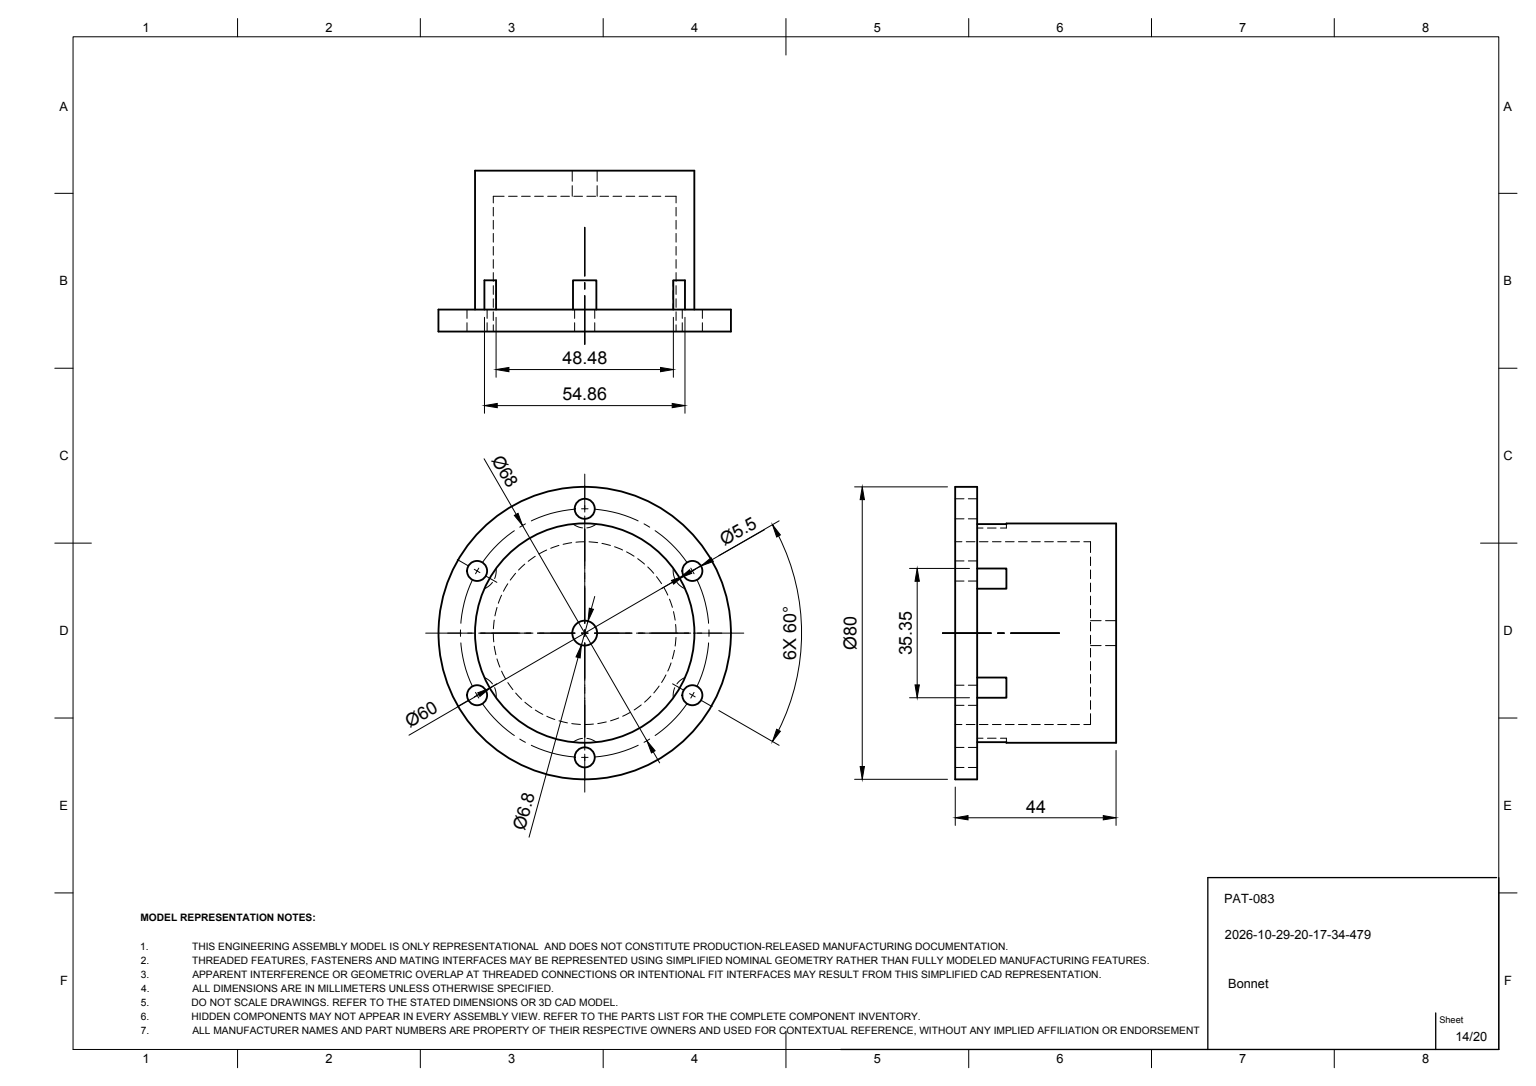
ISO-10303-21;
HEADER;
/* Generated by software containing ST-Developer
 * from STEP Tools, Inc. (www.steptools.com) 
 */

FILE_DESCRIPTION(
/* description */ ('PAT-083'),
/* implementation_level */ '2;1');

FILE_NAME(
/* name */ 'Bonnet.step',
/* time_stamp */ '2026-10-29T20:18:00-07:00',
/* author */ (''),
/* organization */ (''),
/* preprocessor_version */ 'ST-DEVELOPER v20.2',
/* originating_system */ 'Autodesk Translation Framework v15.17.0.0',
/* authorisation */ '');

FILE_SCHEMA (('AUTOMOTIVE_DESIGN { 1 0 10303 214 3 1 1 }'));
ENDSEC;

DATA;
#10=MECHANICAL_DESIGN_GEOMETRIC_PRESENTATION_REPRESENTATION('',(#240),#8428);
#192=SHAPE_REPRESENTATION_RELATIONSHIP('SRR','None',#8526,#216);
#216=ADVANCED_BREP_SHAPE_REPRESENTATION('',(#264),#8415);
#240=STYLED_ITEM('',(#8698),#264);
#264=MANIFOLD_SOLID_BREP('Body1',#3686);
#324=FACE_BOUND('',#900,.T.);
#325=FACE_BOUND('',#902,.T.);
#326=FACE_BOUND('',#905,.T.);
#327=FACE_BOUND('',#906,.T.);
#328=FACE_BOUND('',#907,.T.);
#329=FACE_BOUND('',#908,.T.);
#330=FACE_BOUND('',#909,.T.);
#331=FACE_BOUND('',#910,.T.);
#332=FACE_BOUND('',#911,.T.);
#333=FACE_BOUND('',#913,.T.);
#334=FACE_BOUND('',#914,.T.);
#335=FACE_BOUND('',#915,.T.);
#336=FACE_BOUND('',#916,.T.);
#337=FACE_BOUND('',#917,.T.);
#338=FACE_BOUND('',#918,.T.);
#339=FACE_BOUND('',#919,.T.);
#411=PLANE('',#4167);
#412=PLANE('',#4175);
#413=PLANE('',#4177);
#414=PLANE('',#4182);
#415=PLANE('',#4187);
#416=PLANE('',#4195);
#417=PLANE('',#4230);
#418=PLANE('',#4231);
#419=PLANE('',#4235);
#420=PLANE('',#4236);
#596=FACE_OUTER_BOUND('',#878,.T.);
#597=FACE_OUTER_BOUND('',#879,.T.);
#598=FACE_OUTER_BOUND('',#880,.T.);
#599=FACE_OUTER_BOUND('',#881,.T.);
#600=FACE_OUTER_BOUND('',#882,.T.);
#601=FACE_OUTER_BOUND('',#883,.T.);
#602=FACE_OUTER_BOUND('',#884,.T.);
#603=FACE_OUTER_BOUND('',#885,.T.);
#604=FACE_OUTER_BOUND('',#886,.T.);
#605=FACE_OUTER_BOUND('',#887,.T.);
#606=FACE_OUTER_BOUND('',#888,.T.);
#607=FACE_OUTER_BOUND('',#889,.T.);
#608=FACE_OUTER_BOUND('',#890,.T.);
#609=FACE_OUTER_BOUND('',#891,.T.);
#610=FACE_OUTER_BOUND('',#892,.T.);
#611=FACE_OUTER_BOUND('',#893,.T.);
#612=FACE_OUTER_BOUND('',#894,.T.);
#613=FACE_OUTER_BOUND('',#895,.T.);
#614=FACE_OUTER_BOUND('',#896,.T.);
#615=FACE_OUTER_BOUND('',#897,.T.);
#616=FACE_OUTER_BOUND('',#898,.T.);
#617=FACE_OUTER_BOUND('',#899,.T.);
#618=FACE_OUTER_BOUND('',#901,.T.);
#619=FACE_OUTER_BOUND('',#903,.T.);
#620=FACE_OUTER_BOUND('',#904,.T.);
#621=FACE_OUTER_BOUND('',#912,.T.);
#878=EDGE_LOOP('',(#2828,#2829));
#879=EDGE_LOOP('',(#2830,#2831,#2832,#2833));
#880=EDGE_LOOP('',(#2834,#2835,#2836,#2837));
#881=EDGE_LOOP('',(#2838,#2839));
#882=EDGE_LOOP('',(#2840,#2841));
#883=EDGE_LOOP('',(#2842,#2843,#2844,#2845));
#884=EDGE_LOOP('',(#2846,#2847));
#885=EDGE_LOOP('',(#2848,#2849,#2850,#2851));
#886=EDGE_LOOP('',(#2852,#2853));
#887=EDGE_LOOP('',(#2854,#2855,#2856,#2857));
#888=EDGE_LOOP('',(#2858,#2859,#2860,#2861));
#889=EDGE_LOOP('',(#2862,#2863));
#890=EDGE_LOOP('',(#2864,#2865,#2866,#2867,#2868,#2869,#2870,#2871,#2872,
#2873,#2874,#2875,#2876,#2877,#2878,#2879,#2880,#2881,#2882,#2883,#2884,
#2885,#2886,#2887,#2888,#2889,#2890,#2891));
#891=EDGE_LOOP('',(#2892,#2893,#2894,#2895));
#892=EDGE_LOOP('',(#2896,#2897,#2898,#2899));
#893=EDGE_LOOP('',(#2900,#2901,#2902,#2903));
#894=EDGE_LOOP('',(#2904,#2905,#2906,#2907));
#895=EDGE_LOOP('',(#2908,#2909,#2910,#2911));
#896=EDGE_LOOP('',(#2912,#2913,#2914,#2915));
#897=EDGE_LOOP('',(#2916,#2917,#2918,#2919));
#898=EDGE_LOOP('',(#2920,#2921,#2922,#2923));
#899=EDGE_LOOP('',(#2924));
#900=EDGE_LOOP('',(#2925));
#901=EDGE_LOOP('',(#2926));
#902=EDGE_LOOP('',(#2927));
#903=EDGE_LOOP('',(#2928,#2929,#2930,#2931));
#904=EDGE_LOOP('',(#2932));
#905=EDGE_LOOP('',(#2933));
#906=EDGE_LOOP('',(#2934));
#907=EDGE_LOOP('',(#2935));
#908=EDGE_LOOP('',(#2936));
#909=EDGE_LOOP('',(#2937));
#910=EDGE_LOOP('',(#2938));
#911=EDGE_LOOP('',(#2939,#2940,#2941,#2942,#2943,#2944,#2945,#2946,#2947,
#2948,#2949,#2950,#2951));
#912=EDGE_LOOP('',(#2952));
#913=EDGE_LOOP('',(#2953));
#914=EDGE_LOOP('',(#2954));
#915=EDGE_LOOP('',(#2955));
#916=EDGE_LOOP('',(#2956));
#917=EDGE_LOOP('',(#2957));
#918=EDGE_LOOP('',(#2958));
#919=EDGE_LOOP('',(#2959));
#1129=LINE('',#6913,#1373);
#1130=LINE('',#6916,#1374);
#1131=LINE('',#6920,#1375);
#1132=LINE('',#6924,#1376);
#1133=LINE('',#6935,#1377);
#1134=LINE('',#6938,#1378);
#1135=LINE('',#6946,#1379);
#1136=LINE('',#6949,#1380);
#1137=LINE('',#6957,#1381);
#1138=LINE('',#6960,#1382);
#1139=LINE('',#6964,#1383);
#1140=LINE('',#6968,#1384);
#1141=LINE('',#6976,#1385);
#1142=LINE('',#6988,#1386);
#1143=LINE('',#6994,#1387);
#1144=LINE('',#7000,#1388);
#1145=LINE('',#7006,#1389);
#1146=LINE('',#7012,#1390);
#1147=LINE('',#7018,#1391);
#1148=LINE('',#7024,#1392);
#1149=LINE('',#7030,#1393);
#1150=LINE('',#7038,#1394);
#1373=VECTOR('',#4933,1.);
#1374=VECTOR('',#4936,1.);
#1375=VECTOR('',#4939,1.);
#1376=VECTOR('',#4942,1.);
#1377=VECTOR('',#4957,1.);
#1378=VECTOR('',#4960,1.);
#1379=VECTOR('',#4969,1.);
#1380=VECTOR('',#4972,1.);
#1381=VECTOR('',#4981,1.);
#1382=VECTOR('',#4984,1.);
#1383=VECTOR('',#4987,1.);
#1384=VECTOR('',#4990,1.);
#1385=VECTOR('',#5001,3.);
#1386=VECTOR('',#5020,0.275);
#1387=VECTOR('',#5027,0.275);
#1388=VECTOR('',#5034,0.275);
#1389=VECTOR('',#5041,0.275);
#1390=VECTOR('',#5048,0.275);
#1391=VECTOR('',#5055,0.275);
#1392=VECTOR('',#5062,0.34);
#1393=VECTOR('',#5069,2.5);
#1394=VECTOR('',#5080,4.);
#1618=CIRCLE('',#4168,3.);
#1619=CIRCLE('',#4169,0.525);
#1620=CIRCLE('',#4171,0.525);
#1621=CIRCLE('',#4173,0.525);
#1622=CIRCLE('',#4174,0.525);
#1623=CIRCLE('',#4176,3.);
#1624=CIRCLE('',#4178,3.);
#1625=CIRCLE('',#4179,0.525);
#1626=CIRCLE('',#4181,0.525);
#1627=CIRCLE('',#4183,3.);
#1628=CIRCLE('',#4184,0.525);
#1629=CIRCLE('',#4186,0.525);
#1630=CIRCLE('',#4188,3.);
#1631=CIRCLE('',#4189,0.525);
#1632=CIRCLE('',#4191,0.525);
#1633=CIRCLE('',#4193,0.525);
#1634=CIRCLE('',#4194,0.525);
#1635=CIRCLE('',#4196,3.);
#1636=CIRCLE('',#4198,3.);
#1637=CIRCLE('',#4199,3.);
#1638=CIRCLE('',#4200,3.);
#1639=CIRCLE('',#4201,3.);
#1640=CIRCLE('',#4202,3.);
#1641=CIRCLE('',#4203,3.);
#1642=CIRCLE('',#4204,3.);
#1643=CIRCLE('',#4205,3.);
#1644=CIRCLE('',#4207,0.275);
#1645=CIRCLE('',#4208,0.275);
#1646=CIRCLE('',#4210,0.275);
#1647=CIRCLE('',#4211,0.275);
#1648=CIRCLE('',#4213,0.275);
#1649=CIRCLE('',#4214,0.275);
#1650=CIRCLE('',#4216,0.275);
#1651=CIRCLE('',#4217,0.275);
#1652=CIRCLE('',#4219,0.275);
#1653=CIRCLE('',#4220,0.275);
#1654=CIRCLE('',#4222,0.275);
#1655=CIRCLE('',#4223,0.275);
#1656=CIRCLE('',#4225,0.34);
#1657=CIRCLE('',#4226,0.34);
#1658=CIRCLE('',#4228,2.5);
#1659=CIRCLE('',#4229,2.5);
#1660=CIRCLE('',#4233,4.);
#1661=CIRCLE('',#4234,4.);
#1831=VERTEX_POINT('',#6907);
#1832=VERTEX_POINT('',#6908);
#1833=VERTEX_POINT('',#6912);
#1834=VERTEX_POINT('',#6914);
#1835=VERTEX_POINT('',#6918);
#1836=VERTEX_POINT('',#6919);
#1837=VERTEX_POINT('',#6921);
#1838=VERTEX_POINT('',#6923);
#1839=VERTEX_POINT('',#6929);
#1840=VERTEX_POINT('',#6930);
#1841=VERTEX_POINT('',#6934);
#1842=VERTEX_POINT('',#6936);
#1843=VERTEX_POINT('',#6940);
#1844=VERTEX_POINT('',#6941);
#1845=VERTEX_POINT('',#6945);
#1846=VERTEX_POINT('',#6947);
#1847=VERTEX_POINT('',#6951);
#1848=VERTEX_POINT('',#6952);
#1849=VERTEX_POINT('',#6956);
#1850=VERTEX_POINT('',#6958);
#1851=VERTEX_POINT('',#6962);
#1852=VERTEX_POINT('',#6963);
#1853=VERTEX_POINT('',#6965);
#1854=VERTEX_POINT('',#6967);
#1855=VERTEX_POINT('',#6973);
#1856=VERTEX_POINT('',#6975);
#1857=VERTEX_POINT('',#6985);
#1858=VERTEX_POINT('',#6987);
#1859=VERTEX_POINT('',#6991);
#1860=VERTEX_POINT('',#6993);
#1861=VERTEX_POINT('',#6997);
#1862=VERTEX_POINT('',#6999);
#1863=VERTEX_POINT('',#7003);
#1864=VERTEX_POINT('',#7005);
#1865=VERTEX_POINT('',#7009);
#1866=VERTEX_POINT('',#7011);
#1867=VERTEX_POINT('',#7015);
#1868=VERTEX_POINT('',#7017);
#1869=VERTEX_POINT('',#7021);
#1870=VERTEX_POINT('',#7023);
#1871=VERTEX_POINT('',#7027);
#1872=VERTEX_POINT('',#7029);
#1873=VERTEX_POINT('',#7035);
#1874=VERTEX_POINT('',#7037);
#2190=EDGE_CURVE('',#1831,#1832,#1618,.T.);
#2191=EDGE_CURVE('',#1832,#1831,#1619,.T.);
#2192=EDGE_CURVE('',#1833,#1831,#1129,.T.);
#2193=EDGE_CURVE('',#1834,#1833,#1620,.T.);
#2194=EDGE_CURVE('',#1832,#1834,#1130,.T.);
#2195=EDGE_CURVE('',#1835,#1836,#1131,.T.);
#2196=EDGE_CURVE('',#1835,#1837,#1621,.T.);
#2197=EDGE_CURVE('',#1838,#1837,#1132,.T.);
#2198=EDGE_CURVE('',#1836,#1838,#1622,.T.);
#2199=EDGE_CURVE('',#1837,#1835,#1623,.T.);
#2200=EDGE_CURVE('',#1839,#1840,#1624,.T.);
#2201=EDGE_CURVE('',#1840,#1839,#1625,.T.);
#2202=EDGE_CURVE('',#1841,#1839,#1133,.T.);
#2203=EDGE_CURVE('',#1842,#1841,#1626,.T.);
#2204=EDGE_CURVE('',#1840,#1842,#1134,.T.);
#2205=EDGE_CURVE('',#1843,#1844,#1627,.T.);
#2206=EDGE_CURVE('',#1844,#1843,#1628,.T.);
#2207=EDGE_CURVE('',#1845,#1843,#1135,.T.);
#2208=EDGE_CURVE('',#1846,#1845,#1629,.T.);
#2209=EDGE_CURVE('',#1844,#1846,#1136,.T.);
#2210=EDGE_CURVE('',#1847,#1848,#1630,.T.);
#2211=EDGE_CURVE('',#1848,#1847,#1631,.T.);
#2212=EDGE_CURVE('',#1849,#1847,#1137,.T.);
#2213=EDGE_CURVE('',#1850,#1849,#1632,.T.);
#2214=EDGE_CURVE('',#1848,#1850,#1138,.T.);
#2215=EDGE_CURVE('',#1851,#1852,#1139,.T.);
#2216=EDGE_CURVE('',#1851,#1853,#1633,.T.);
#2217=EDGE_CURVE('',#1854,#1853,#1140,.T.);
#2218=EDGE_CURVE('',#1852,#1854,#1634,.T.);
#2219=EDGE_CURVE('',#1853,#1851,#1635,.T.);
#2220=EDGE_CURVE('',#1855,#1855,#1636,.T.);
#2221=EDGE_CURVE('',#1855,#1856,#1141,.T.);
#2222=EDGE_CURVE('',#1849,#1856,#1637,.T.);
#2223=EDGE_CURVE('',#1833,#1850,#1638,.T.);
#2224=EDGE_CURVE('',#1854,#1834,#1639,.T.);
#2225=EDGE_CURVE('',#1838,#1852,#1640,.T.);
#2226=EDGE_CURVE('',#1841,#1836,#1641,.T.);
#2227=EDGE_CURVE('',#1845,#1842,#1642,.T.);
#2228=EDGE_CURVE('',#1856,#1846,#1643,.T.);
#2229=EDGE_CURVE('',#1857,#1857,#1644,.T.);
#2230=EDGE_CURVE('',#1857,#1858,#1142,.T.);
#2231=EDGE_CURVE('',#1858,#1858,#1645,.T.);
#2232=EDGE_CURVE('',#1859,#1859,#1646,.T.);
#2233=EDGE_CURVE('',#1859,#1860,#1143,.T.);
#2234=EDGE_CURVE('',#1860,#1860,#1647,.T.);
#2235=EDGE_CURVE('',#1861,#1861,#1648,.T.);
#2236=EDGE_CURVE('',#1861,#1862,#1144,.T.);
#2237=EDGE_CURVE('',#1862,#1862,#1649,.T.);
#2238=EDGE_CURVE('',#1863,#1863,#1650,.T.);
#2239=EDGE_CURVE('',#1863,#1864,#1145,.T.);
#2240=EDGE_CURVE('',#1864,#1864,#1651,.T.);
#2241=EDGE_CURVE('',#1865,#1865,#1652,.T.);
#2242=EDGE_CURVE('',#1865,#1866,#1146,.T.);
#2243=EDGE_CURVE('',#1866,#1866,#1653,.T.);
#2244=EDGE_CURVE('',#1867,#1867,#1654,.T.);
#2245=EDGE_CURVE('',#1867,#1868,#1147,.T.);
#2246=EDGE_CURVE('',#1868,#1868,#1655,.T.);
#2247=EDGE_CURVE('',#1869,#1869,#1656,.T.);
#2248=EDGE_CURVE('',#1869,#1870,#1148,.T.);
#2249=EDGE_CURVE('',#1870,#1870,#1657,.T.);
#2250=EDGE_CURVE('',#1871,#1871,#1658,.T.);
#2251=EDGE_CURVE('',#1871,#1872,#1149,.T.);
#2252=EDGE_CURVE('',#1872,#1872,#1659,.T.);
#2253=EDGE_CURVE('',#1873,#1873,#1660,.T.);
#2254=EDGE_CURVE('',#1873,#1874,#1150,.T.);
#2255=EDGE_CURVE('',#1874,#1874,#1661,.T.);
#2828=ORIENTED_EDGE('',*,*,#2190,.F.);
#2829=ORIENTED_EDGE('',*,*,#2191,.F.);
#2830=ORIENTED_EDGE('',*,*,#2192,.F.);
#2831=ORIENTED_EDGE('',*,*,#2193,.F.);
#2832=ORIENTED_EDGE('',*,*,#2194,.F.);
#2833=ORIENTED_EDGE('',*,*,#2191,.T.);
#2834=ORIENTED_EDGE('',*,*,#2195,.F.);
#2835=ORIENTED_EDGE('',*,*,#2196,.T.);
#2836=ORIENTED_EDGE('',*,*,#2197,.F.);
#2837=ORIENTED_EDGE('',*,*,#2198,.F.);
#2838=ORIENTED_EDGE('',*,*,#2199,.F.);
#2839=ORIENTED_EDGE('',*,*,#2196,.F.);
#2840=ORIENTED_EDGE('',*,*,#2200,.F.);
#2841=ORIENTED_EDGE('',*,*,#2201,.F.);
#2842=ORIENTED_EDGE('',*,*,#2202,.F.);
#2843=ORIENTED_EDGE('',*,*,#2203,.F.);
#2844=ORIENTED_EDGE('',*,*,#2204,.F.);
#2845=ORIENTED_EDGE('',*,*,#2201,.T.);
#2846=ORIENTED_EDGE('',*,*,#2205,.F.);
#2847=ORIENTED_EDGE('',*,*,#2206,.F.);
#2848=ORIENTED_EDGE('',*,*,#2207,.F.);
#2849=ORIENTED_EDGE('',*,*,#2208,.F.);
#2850=ORIENTED_EDGE('',*,*,#2209,.F.);
#2851=ORIENTED_EDGE('',*,*,#2206,.T.);
#2852=ORIENTED_EDGE('',*,*,#2210,.F.);
#2853=ORIENTED_EDGE('',*,*,#2211,.F.);
#2854=ORIENTED_EDGE('',*,*,#2212,.F.);
#2855=ORIENTED_EDGE('',*,*,#2213,.F.);
#2856=ORIENTED_EDGE('',*,*,#2214,.F.);
#2857=ORIENTED_EDGE('',*,*,#2211,.T.);
#2858=ORIENTED_EDGE('',*,*,#2215,.F.);
#2859=ORIENTED_EDGE('',*,*,#2216,.T.);
#2860=ORIENTED_EDGE('',*,*,#2217,.F.);
#2861=ORIENTED_EDGE('',*,*,#2218,.F.);
#2862=ORIENTED_EDGE('',*,*,#2219,.F.);
#2863=ORIENTED_EDGE('',*,*,#2216,.F.);
#2864=ORIENTED_EDGE('',*,*,#2220,.F.);
#2865=ORIENTED_EDGE('',*,*,#2221,.T.);
#2866=ORIENTED_EDGE('',*,*,#2222,.F.);
#2867=ORIENTED_EDGE('',*,*,#2212,.T.);
#2868=ORIENTED_EDGE('',*,*,#2210,.T.);
#2869=ORIENTED_EDGE('',*,*,#2214,.T.);
#2870=ORIENTED_EDGE('',*,*,#2223,.F.);
#2871=ORIENTED_EDGE('',*,*,#2192,.T.);
#2872=ORIENTED_EDGE('',*,*,#2190,.T.);
#2873=ORIENTED_EDGE('',*,*,#2194,.T.);
#2874=ORIENTED_EDGE('',*,*,#2224,.F.);
#2875=ORIENTED_EDGE('',*,*,#2217,.T.);
#2876=ORIENTED_EDGE('',*,*,#2219,.T.);
#2877=ORIENTED_EDGE('',*,*,#2215,.T.);
#2878=ORIENTED_EDGE('',*,*,#2225,.F.);
#2879=ORIENTED_EDGE('',*,*,#2197,.T.);
#2880=ORIENTED_EDGE('',*,*,#2199,.T.);
#2881=ORIENTED_EDGE('',*,*,#2195,.T.);
#2882=ORIENTED_EDGE('',*,*,#2226,.F.);
#2883=ORIENTED_EDGE('',*,*,#2202,.T.);
#2884=ORIENTED_EDGE('',*,*,#2200,.T.);
#2885=ORIENTED_EDGE('',*,*,#2204,.T.);
#2886=ORIENTED_EDGE('',*,*,#2227,.F.);
#2887=ORIENTED_EDGE('',*,*,#2207,.T.);
#2888=ORIENTED_EDGE('',*,*,#2205,.T.);
#2889=ORIENTED_EDGE('',*,*,#2209,.T.);
#2890=ORIENTED_EDGE('',*,*,#2228,.F.);
#2891=ORIENTED_EDGE('',*,*,#2221,.F.);
#2892=ORIENTED_EDGE('',*,*,#2229,.F.);
#2893=ORIENTED_EDGE('',*,*,#2230,.T.);
#2894=ORIENTED_EDGE('',*,*,#2231,.F.);
#2895=ORIENTED_EDGE('',*,*,#2230,.F.);
#2896=ORIENTED_EDGE('',*,*,#2232,.F.);
#2897=ORIENTED_EDGE('',*,*,#2233,.T.);
#2898=ORIENTED_EDGE('',*,*,#2234,.F.);
#2899=ORIENTED_EDGE('',*,*,#2233,.F.);
#2900=ORIENTED_EDGE('',*,*,#2235,.F.);
#2901=ORIENTED_EDGE('',*,*,#2236,.T.);
#2902=ORIENTED_EDGE('',*,*,#2237,.F.);
#2903=ORIENTED_EDGE('',*,*,#2236,.F.);
#2904=ORIENTED_EDGE('',*,*,#2238,.F.);
#2905=ORIENTED_EDGE('',*,*,#2239,.T.);
#2906=ORIENTED_EDGE('',*,*,#2240,.F.);
#2907=ORIENTED_EDGE('',*,*,#2239,.F.);
#2908=ORIENTED_EDGE('',*,*,#2241,.F.);
#2909=ORIENTED_EDGE('',*,*,#2242,.T.);
#2910=ORIENTED_EDGE('',*,*,#2243,.F.);
#2911=ORIENTED_EDGE('',*,*,#2242,.F.);
#2912=ORIENTED_EDGE('',*,*,#2244,.F.);
#2913=ORIENTED_EDGE('',*,*,#2245,.T.);
#2914=ORIENTED_EDGE('',*,*,#2246,.F.);
#2915=ORIENTED_EDGE('',*,*,#2245,.F.);
#2916=ORIENTED_EDGE('',*,*,#2247,.F.);
#2917=ORIENTED_EDGE('',*,*,#2248,.T.);
#2918=ORIENTED_EDGE('',*,*,#2249,.F.);
#2919=ORIENTED_EDGE('',*,*,#2248,.F.);
#2920=ORIENTED_EDGE('',*,*,#2250,.F.);
#2921=ORIENTED_EDGE('',*,*,#2251,.T.);
#2922=ORIENTED_EDGE('',*,*,#2252,.T.);
#2923=ORIENTED_EDGE('',*,*,#2251,.F.);
#2924=ORIENTED_EDGE('',*,*,#2252,.F.);
#2925=ORIENTED_EDGE('',*,*,#2247,.T.);
#2926=ORIENTED_EDGE('',*,*,#2220,.T.);
#2927=ORIENTED_EDGE('',*,*,#2249,.T.);
#2928=ORIENTED_EDGE('',*,*,#2253,.F.);
#2929=ORIENTED_EDGE('',*,*,#2254,.T.);
#2930=ORIENTED_EDGE('',*,*,#2255,.T.);
#2931=ORIENTED_EDGE('',*,*,#2254,.F.);
#2932=ORIENTED_EDGE('',*,*,#2253,.T.);
#2933=ORIENTED_EDGE('',*,*,#2231,.T.);
#2934=ORIENTED_EDGE('',*,*,#2234,.T.);
#2935=ORIENTED_EDGE('',*,*,#2237,.T.);
#2936=ORIENTED_EDGE('',*,*,#2240,.T.);
#2937=ORIENTED_EDGE('',*,*,#2243,.T.);
#2938=ORIENTED_EDGE('',*,*,#2246,.T.);
#2939=ORIENTED_EDGE('',*,*,#2223,.T.);
#2940=ORIENTED_EDGE('',*,*,#2213,.T.);
#2941=ORIENTED_EDGE('',*,*,#2222,.T.);
#2942=ORIENTED_EDGE('',*,*,#2228,.T.);
#2943=ORIENTED_EDGE('',*,*,#2208,.T.);
#2944=ORIENTED_EDGE('',*,*,#2227,.T.);
#2945=ORIENTED_EDGE('',*,*,#2203,.T.);
#2946=ORIENTED_EDGE('',*,*,#2226,.T.);
#2947=ORIENTED_EDGE('',*,*,#2198,.T.);
#2948=ORIENTED_EDGE('',*,*,#2225,.T.);
#2949=ORIENTED_EDGE('',*,*,#2218,.T.);
#2950=ORIENTED_EDGE('',*,*,#2224,.T.);
#2951=ORIENTED_EDGE('',*,*,#2193,.T.);
#2952=ORIENTED_EDGE('',*,*,#2255,.F.);
#2953=ORIENTED_EDGE('',*,*,#2250,.T.);
#2954=ORIENTED_EDGE('',*,*,#2244,.T.);
#2955=ORIENTED_EDGE('',*,*,#2241,.T.);
#2956=ORIENTED_EDGE('',*,*,#2238,.T.);
#2957=ORIENTED_EDGE('',*,*,#2235,.T.);
#2958=ORIENTED_EDGE('',*,*,#2232,.T.);
#2959=ORIENTED_EDGE('',*,*,#2229,.T.);
#3409=CYLINDRICAL_SURFACE('',#4170,0.525);
#3410=CYLINDRICAL_SURFACE('',#4172,0.525);
#3411=CYLINDRICAL_SURFACE('',#4180,0.525);
#3412=CYLINDRICAL_SURFACE('',#4185,0.525);
#3413=CYLINDRICAL_SURFACE('',#4190,0.525);
#3414=CYLINDRICAL_SURFACE('',#4192,0.525);
#3415=CYLINDRICAL_SURFACE('',#4197,3.);
#3416=CYLINDRICAL_SURFACE('',#4206,0.275);
#3417=CYLINDRICAL_SURFACE('',#4209,0.275);
#3418=CYLINDRICAL_SURFACE('',#4212,0.275);
#3419=CYLINDRICAL_SURFACE('',#4215,0.275);
#3420=CYLINDRICAL_SURFACE('',#4218,0.275);
#3421=CYLINDRICAL_SURFACE('',#4221,0.275);
#3422=CYLINDRICAL_SURFACE('',#4224,0.34);
#3423=CYLINDRICAL_SURFACE('',#4227,2.5);
#3424=CYLINDRICAL_SURFACE('',#4232,4.);
#3543=ADVANCED_FACE('',(#596),#411,.F.);
#3544=ADVANCED_FACE('',(#597),#3409,.F.);
#3545=ADVANCED_FACE('',(#598),#3410,.F.);
#3546=ADVANCED_FACE('',(#599),#412,.F.);
#3547=ADVANCED_FACE('',(#600),#413,.F.);
#3548=ADVANCED_FACE('',(#601),#3411,.F.);
#3549=ADVANCED_FACE('',(#602),#414,.F.);
#3550=ADVANCED_FACE('',(#603),#3412,.F.);
#3551=ADVANCED_FACE('',(#604),#415,.F.);
#3552=ADVANCED_FACE('',(#605),#3413,.F.);
#3553=ADVANCED_FACE('',(#606),#3414,.F.);
#3554=ADVANCED_FACE('',(#607),#416,.F.);
#3555=ADVANCED_FACE('',(#608),#3415,.T.);
#3556=ADVANCED_FACE('',(#609),#3416,.F.);
#3557=ADVANCED_FACE('',(#610),#3417,.F.);
#3558=ADVANCED_FACE('',(#611),#3418,.F.);
#3559=ADVANCED_FACE('',(#612),#3419,.F.);
#3560=ADVANCED_FACE('',(#613),#3420,.F.);
#3561=ADVANCED_FACE('',(#614),#3421,.F.);
#3562=ADVANCED_FACE('',(#615),#3422,.F.);
#3563=ADVANCED_FACE('',(#616),#3423,.F.);
#3564=ADVANCED_FACE('',(#617,#324),#417,.F.);
#3565=ADVANCED_FACE('',(#618,#325),#418,.T.);
#3566=ADVANCED_FACE('',(#619),#3424,.T.);
#3567=ADVANCED_FACE('',(#620,#326,#327,#328,#329,#330,#331,#332),#419,.T.);
#3568=ADVANCED_FACE('',(#621,#333,#334,#335,#336,#337,#338,#339),#420,.F.);
#3686=CLOSED_SHELL('',(#3543,#3544,#3545,#3546,#3547,#3548,#3549,#3550,
#3551,#3552,#3553,#3554,#3555,#3556,#3557,#3558,#3559,#3560,#3561,#3562,
#3563,#3564,#3565,#3566,#3567,#3568));
#4166=AXIS2_PLACEMENT_3D('',#6905,#4923,#4924);
#4167=AXIS2_PLACEMENT_3D('',#6906,#4925,#4926);
#4168=AXIS2_PLACEMENT_3D('',#6909,#4927,#4928);
#4169=AXIS2_PLACEMENT_3D('',#6910,#4929,#4930);
#4170=AXIS2_PLACEMENT_3D('',#6911,#4931,#4932);
#4171=AXIS2_PLACEMENT_3D('',#6915,#4934,#4935);
#4172=AXIS2_PLACEMENT_3D('',#6917,#4937,#4938);
#4173=AXIS2_PLACEMENT_3D('',#6922,#4940,#4941);
#4174=AXIS2_PLACEMENT_3D('',#6925,#4943,#4944);
#4175=AXIS2_PLACEMENT_3D('',#6926,#4945,#4946);
#4176=AXIS2_PLACEMENT_3D('',#6927,#4947,#4948);
#4177=AXIS2_PLACEMENT_3D('',#6928,#4949,#4950);
#4178=AXIS2_PLACEMENT_3D('',#6931,#4951,#4952);
#4179=AXIS2_PLACEMENT_3D('',#6932,#4953,#4954);
#4180=AXIS2_PLACEMENT_3D('',#6933,#4955,#4956);
#4181=AXIS2_PLACEMENT_3D('',#6937,#4958,#4959);
#4182=AXIS2_PLACEMENT_3D('',#6939,#4961,#4962);
#4183=AXIS2_PLACEMENT_3D('',#6942,#4963,#4964);
#4184=AXIS2_PLACEMENT_3D('',#6943,#4965,#4966);
#4185=AXIS2_PLACEMENT_3D('',#6944,#4967,#4968);
#4186=AXIS2_PLACEMENT_3D('',#6948,#4970,#4971);
#4187=AXIS2_PLACEMENT_3D('',#6950,#4973,#4974);
#4188=AXIS2_PLACEMENT_3D('',#6953,#4975,#4976);
#4189=AXIS2_PLACEMENT_3D('',#6954,#4977,#4978);
#4190=AXIS2_PLACEMENT_3D('',#6955,#4979,#4980);
#4191=AXIS2_PLACEMENT_3D('',#6959,#4982,#4983);
#4192=AXIS2_PLACEMENT_3D('',#6961,#4985,#4986);
#4193=AXIS2_PLACEMENT_3D('',#6966,#4988,#4989);
#4194=AXIS2_PLACEMENT_3D('',#6969,#4991,#4992);
#4195=AXIS2_PLACEMENT_3D('',#6970,#4993,#4994);
#4196=AXIS2_PLACEMENT_3D('',#6971,#4995,#4996);
#4197=AXIS2_PLACEMENT_3D('',#6972,#4997,#4998);
#4198=AXIS2_PLACEMENT_3D('',#6974,#4999,#5000);
#4199=AXIS2_PLACEMENT_3D('',#6977,#5002,#5003);
#4200=AXIS2_PLACEMENT_3D('',#6978,#5004,#5005);
#4201=AXIS2_PLACEMENT_3D('',#6979,#5006,#5007);
#4202=AXIS2_PLACEMENT_3D('',#6980,#5008,#5009);
#4203=AXIS2_PLACEMENT_3D('',#6981,#5010,#5011);
#4204=AXIS2_PLACEMENT_3D('',#6982,#5012,#5013);
#4205=AXIS2_PLACEMENT_3D('',#6983,#5014,#5015);
#4206=AXIS2_PLACEMENT_3D('',#6984,#5016,#5017);
#4207=AXIS2_PLACEMENT_3D('',#6986,#5018,#5019);
#4208=AXIS2_PLACEMENT_3D('',#6989,#5021,#5022);
#4209=AXIS2_PLACEMENT_3D('',#6990,#5023,#5024);
#4210=AXIS2_PLACEMENT_3D('',#6992,#5025,#5026);
#4211=AXIS2_PLACEMENT_3D('',#6995,#5028,#5029);
#4212=AXIS2_PLACEMENT_3D('',#6996,#5030,#5031);
#4213=AXIS2_PLACEMENT_3D('',#6998,#5032,#5033);
#4214=AXIS2_PLACEMENT_3D('',#7001,#5035,#5036);
#4215=AXIS2_PLACEMENT_3D('',#7002,#5037,#5038);
#4216=AXIS2_PLACEMENT_3D('',#7004,#5039,#5040);
#4217=AXIS2_PLACEMENT_3D('',#7007,#5042,#5043);
#4218=AXIS2_PLACEMENT_3D('',#7008,#5044,#5045);
#4219=AXIS2_PLACEMENT_3D('',#7010,#5046,#5047);
#4220=AXIS2_PLACEMENT_3D('',#7013,#5049,#5050);
#4221=AXIS2_PLACEMENT_3D('',#7014,#5051,#5052);
#4222=AXIS2_PLACEMENT_3D('',#7016,#5053,#5054);
#4223=AXIS2_PLACEMENT_3D('',#7019,#5056,#5057);
#4224=AXIS2_PLACEMENT_3D('',#7020,#5058,#5059);
#4225=AXIS2_PLACEMENT_3D('',#7022,#5060,#5061);
#4226=AXIS2_PLACEMENT_3D('',#7025,#5063,#5064);
#4227=AXIS2_PLACEMENT_3D('',#7026,#5065,#5066);
#4228=AXIS2_PLACEMENT_3D('',#7028,#5067,#5068);
#4229=AXIS2_PLACEMENT_3D('',#7031,#5070,#5071);
#4230=AXIS2_PLACEMENT_3D('',#7032,#5072,#5073);
#4231=AXIS2_PLACEMENT_3D('',#7033,#5074,#5075);
#4232=AXIS2_PLACEMENT_3D('',#7034,#5076,#5077);
#4233=AXIS2_PLACEMENT_3D('',#7036,#5078,#5079);
#4234=AXIS2_PLACEMENT_3D('',#7039,#5081,#5082);
#4235=AXIS2_PLACEMENT_3D('',#7040,#5083,#5084);
#4236=AXIS2_PLACEMENT_3D('',#7041,#5085,#5086);
#4923=DIRECTION('axis',(0.,0.,1.));
#4924=DIRECTION('refdir',(1.,0.,0.));
#4925=DIRECTION('center_axis',(0.,0.,1.));
#4926=DIRECTION('ref_axis',(1.,0.,0.));
#4927=DIRECTION('center_axis',(0.,0.,1.));
#4928=DIRECTION('ref_axis',(1.,0.,0.));
#4929=DIRECTION('center_axis',(0.,0.,1.));
#4930=DIRECTION('ref_axis',(1.,0.,0.));
#4931=DIRECTION('center_axis',(0.,0.,1.));
#4932=DIRECTION('ref_axis',(1.,0.,0.));
#4933=DIRECTION('',(0.,0.,1.));
#4934=DIRECTION('center_axis',(0.,0.,1.));
#4935=DIRECTION('ref_axis',(1.,0.,0.));
#4936=DIRECTION('',(0.,0.,-1.));
#4937=DIRECTION('center_axis',(0.,0.,1.));
#4938=DIRECTION('ref_axis',(-0.866025403784439,-0.5,0.));
#4939=DIRECTION('',(0.,0.,-1.));
#4940=DIRECTION('center_axis',(0.,0.,1.));
#4941=DIRECTION('ref_axis',(1.,0.,0.));
#4942=DIRECTION('',(0.,0.,1.));
#4943=DIRECTION('center_axis',(0.,0.,1.));
#4944=DIRECTION('ref_axis',(1.,0.,0.));
#4945=DIRECTION('center_axis',(0.,0.,1.));
#4946=DIRECTION('ref_axis',(1.,0.,0.));
#4947=DIRECTION('center_axis',(0.,0.,1.));
#4948=DIRECTION('ref_axis',(1.,0.,0.));
#4949=DIRECTION('center_axis',(0.,0.,1.));
#4950=DIRECTION('ref_axis',(1.,0.,0.));
#4951=DIRECTION('center_axis',(0.,0.,1.));
#4952=DIRECTION('ref_axis',(1.,0.,0.));
#4953=DIRECTION('center_axis',(0.,0.,1.));
#4954=DIRECTION('ref_axis',(1.,0.,0.));
#4955=DIRECTION('center_axis',(0.,0.,1.));
#4956=DIRECTION('ref_axis',(1.,0.,0.));
#4957=DIRECTION('',(0.,0.,1.));
#4958=DIRECTION('center_axis',(0.,0.,1.));
#4959=DIRECTION('ref_axis',(1.,0.,0.));
#4960=DIRECTION('',(0.,0.,-1.));
#4961=DIRECTION('center_axis',(0.,0.,1.));
#4962=DIRECTION('ref_axis',(1.,0.,0.));
#4963=DIRECTION('center_axis',(0.,0.,1.));
#4964=DIRECTION('ref_axis',(1.,0.,0.));
#4965=DIRECTION('center_axis',(0.,0.,1.));
#4966=DIRECTION('ref_axis',(1.,0.,0.));
#4967=DIRECTION('center_axis',(0.,0.,1.));
#4968=DIRECTION('ref_axis',(1.,0.,0.));
#4969=DIRECTION('',(0.,0.,1.));
#4970=DIRECTION('center_axis',(0.,0.,1.));
#4971=DIRECTION('ref_axis',(1.,0.,0.));
#4972=DIRECTION('',(0.,0.,-1.));
#4973=DIRECTION('center_axis',(0.,0.,1.));
#4974=DIRECTION('ref_axis',(1.,0.,0.));
#4975=DIRECTION('center_axis',(0.,0.,1.));
#4976=DIRECTION('ref_axis',(1.,0.,0.));
#4977=DIRECTION('center_axis',(0.,0.,1.));
#4978=DIRECTION('ref_axis',(1.,0.,0.));
#4979=DIRECTION('center_axis',(0.,0.,1.));
#4980=DIRECTION('ref_axis',(1.,0.,0.));
#4981=DIRECTION('',(0.,0.,1.));
#4982=DIRECTION('center_axis',(0.,0.,1.));
#4983=DIRECTION('ref_axis',(1.,0.,0.));
#4984=DIRECTION('',(0.,0.,-1.));
#4985=DIRECTION('center_axis',(0.,0.,1.));
#4986=DIRECTION('ref_axis',(-0.866025403784438,0.5,0.));
#4987=DIRECTION('',(0.,0.,-1.));
#4988=DIRECTION('center_axis',(0.,0.,1.));
#4989=DIRECTION('ref_axis',(1.,0.,0.));
#4990=DIRECTION('',(0.,0.,1.));
#4991=DIRECTION('center_axis',(0.,0.,1.));
#4992=DIRECTION('ref_axis',(1.,0.,0.));
#4993=DIRECTION('center_axis',(0.,0.,1.));
#4994=DIRECTION('ref_axis',(1.,0.,0.));
#4995=DIRECTION('center_axis',(0.,0.,1.));
#4996=DIRECTION('ref_axis',(1.,0.,0.));
#4997=DIRECTION('center_axis',(0.,0.,1.));
#4998=DIRECTION('ref_axis',(1.,0.,0.));
#4999=DIRECTION('center_axis',(0.,0.,1.));
#5000=DIRECTION('ref_axis',(1.,0.,0.));
#5001=DIRECTION('',(0.,0.,-1.));
#5002=DIRECTION('center_axis',(0.,0.,-1.));
#5003=DIRECTION('ref_axis',(1.,0.,0.));
#5004=DIRECTION('center_axis',(0.,0.,-1.));
#5005=DIRECTION('ref_axis',(1.,0.,0.));
#5006=DIRECTION('center_axis',(0.,0.,-1.));
#5007=DIRECTION('ref_axis',(1.,0.,0.));
#5008=DIRECTION('center_axis',(0.,0.,-1.));
#5009=DIRECTION('ref_axis',(1.,0.,0.));
#5010=DIRECTION('center_axis',(0.,0.,-1.));
#5011=DIRECTION('ref_axis',(1.,0.,0.));
#5012=DIRECTION('center_axis',(0.,0.,-1.));
#5013=DIRECTION('ref_axis',(1.,0.,0.));
#5014=DIRECTION('center_axis',(0.,0.,-1.));
#5015=DIRECTION('ref_axis',(1.,0.,0.));
#5016=DIRECTION('center_axis',(0.,0.,1.));
#5017=DIRECTION('ref_axis',(1.,0.,0.));
#5018=DIRECTION('center_axis',(0.,0.,1.));
#5019=DIRECTION('ref_axis',(1.,0.,0.));
#5020=DIRECTION('',(0.,0.,1.));
#5021=DIRECTION('center_axis',(0.,0.,-1.));
#5022=DIRECTION('ref_axis',(1.,0.,0.));
#5023=DIRECTION('center_axis',(0.,0.,1.));
#5024=DIRECTION('ref_axis',(1.,0.,0.));
#5025=DIRECTION('center_axis',(0.,0.,1.));
#5026=DIRECTION('ref_axis',(1.,0.,0.));
#5027=DIRECTION('',(0.,0.,1.));
#5028=DIRECTION('center_axis',(0.,0.,-1.));
#5029=DIRECTION('ref_axis',(1.,0.,0.));
#5030=DIRECTION('center_axis',(0.,0.,1.));
#5031=DIRECTION('ref_axis',(1.,0.,0.));
#5032=DIRECTION('center_axis',(0.,0.,1.));
#5033=DIRECTION('ref_axis',(1.,0.,0.));
#5034=DIRECTION('',(0.,0.,1.));
#5035=DIRECTION('center_axis',(0.,0.,-1.));
#5036=DIRECTION('ref_axis',(1.,0.,0.));
#5037=DIRECTION('center_axis',(0.,0.,1.));
#5038=DIRECTION('ref_axis',(1.,0.,0.));
#5039=DIRECTION('center_axis',(0.,0.,1.));
#5040=DIRECTION('ref_axis',(1.,0.,0.));
#5041=DIRECTION('',(0.,0.,1.));
#5042=DIRECTION('center_axis',(0.,0.,-1.));
#5043=DIRECTION('ref_axis',(1.,0.,0.));
#5044=DIRECTION('center_axis',(0.,0.,1.));
#5045=DIRECTION('ref_axis',(1.,0.,0.));
#5046=DIRECTION('center_axis',(0.,0.,1.));
#5047=DIRECTION('ref_axis',(1.,0.,0.));
#5048=DIRECTION('',(0.,0.,1.));
#5049=DIRECTION('center_axis',(0.,0.,-1.));
#5050=DIRECTION('ref_axis',(1.,0.,0.));
#5051=DIRECTION('center_axis',(0.,0.,1.));
#5052=DIRECTION('ref_axis',(1.,0.,0.));
#5053=DIRECTION('center_axis',(0.,0.,1.));
#5054=DIRECTION('ref_axis',(1.,0.,0.));
#5055=DIRECTION('',(0.,0.,1.));
#5056=DIRECTION('center_axis',(0.,0.,-1.));
#5057=DIRECTION('ref_axis',(1.,0.,0.));
#5058=DIRECTION('center_axis',(0.,0.,1.));
#5059=DIRECTION('ref_axis',(1.,0.,0.));
#5060=DIRECTION('center_axis',(0.,0.,1.));
#5061=DIRECTION('ref_axis',(1.,0.,0.));
#5062=DIRECTION('',(0.,0.,1.));
#5063=DIRECTION('center_axis',(0.,0.,-1.));
#5064=DIRECTION('ref_axis',(1.,0.,0.));
#5065=DIRECTION('center_axis',(0.,0.,1.));
#5066=DIRECTION('ref_axis',(1.,0.,0.));
#5067=DIRECTION('center_axis',(0.,0.,1.));
#5068=DIRECTION('ref_axis',(1.,0.,0.));
#5069=DIRECTION('',(0.,0.,1.));
#5070=DIRECTION('center_axis',(0.,0.,1.));
#5071=DIRECTION('ref_axis',(1.,0.,0.));
#5072=DIRECTION('center_axis',(0.,0.,1.));
#5073=DIRECTION('ref_axis',(1.,0.,0.));
#5074=DIRECTION('center_axis',(0.,0.,1.));
#5075=DIRECTION('ref_axis',(1.,0.,0.));
#5076=DIRECTION('center_axis',(0.,0.,1.));
#5077=DIRECTION('ref_axis',(1.,0.,0.));
#5078=DIRECTION('center_axis',(0.,0.,1.));
#5079=DIRECTION('ref_axis',(1.,0.,0.));
#5080=DIRECTION('',(0.,0.,-1.));
#5081=DIRECTION('center_axis',(0.,0.,1.));
#5082=DIRECTION('ref_axis',(1.,0.,0.));
#5083=DIRECTION('center_axis',(0.,0.,1.));
#5084=DIRECTION('ref_axis',(1.,0.,0.));
#5085=DIRECTION('center_axis',(0.,0.,1.));
#5086=DIRECTION('ref_axis',(1.,0.,0.));
#6905=CARTESIAN_POINT('',(0.,0.,0.));
#6906=CARTESIAN_POINT('Origin',(-6.66133814775094E-16,-3.4,6.5));
#6907=CARTESIAN_POINT('',(-0.318956006072959,-2.98299632352941,6.5));
#6908=CARTESIAN_POINT('',(0.318956006072958,-2.98299632352941,6.5));
#6909=CARTESIAN_POINT('Origin',(0.,0.,6.5));
#6910=CARTESIAN_POINT('Origin',(-6.2456986756515E-16,-3.4,6.5));
#6911=CARTESIAN_POINT('Origin',(-6.2456986756515E-16,-3.4,5.7));
#6912=CARTESIAN_POINT('',(-0.318956006072959,-2.98299632352941,5.7));
#6913=CARTESIAN_POINT('',(-0.318956006072959,-2.98299632352941,5.7));
#6914=CARTESIAN_POINT('',(0.318956006072958,-2.98299632352941,5.7));
#6915=CARTESIAN_POINT('Origin',(-6.2456986756515E-16,-3.4,5.7));
#6916=CARTESIAN_POINT('',(0.318956006072958,-2.98299632352941,5.7));
#6917=CARTESIAN_POINT('Origin',(2.94448637286709,1.7,5.7));
#6918=CARTESIAN_POINT('',(2.42387259253558,1.76772216571351,6.5));
#6919=CARTESIAN_POINT('',(2.42387259253558,1.76772216571351,5.7));
#6920=CARTESIAN_POINT('',(2.42387259253558,1.76772216571351,5.7));
#6921=CARTESIAN_POINT('',(2.74282859860853,1.2152741578159,6.5));
#6922=CARTESIAN_POINT('Origin',(2.94448637286709,1.7,6.5));
#6923=CARTESIAN_POINT('',(2.74282859860853,1.2152741578159,5.7));
#6924=CARTESIAN_POINT('',(2.74282859860853,1.2152741578159,5.7));
#6925=CARTESIAN_POINT('Origin',(2.94448637286709,1.7,5.7));
#6926=CARTESIAN_POINT('Origin',(2.94448637286709,1.7,6.5));
#6927=CARTESIAN_POINT('Origin',(0.,0.,6.5));
#6928=CARTESIAN_POINT('Origin',(2.22044604925031E-16,3.4,6.5));
#6929=CARTESIAN_POINT('',(0.318956006072958,2.98299632352941,6.5));
#6930=CARTESIAN_POINT('',(-0.318956006072958,2.98299632352941,6.5));
#6931=CARTESIAN_POINT('Origin',(0.,0.,6.5));
#6932=CARTESIAN_POINT('Origin',(2.0818995585505E-16,3.4,6.5));
#6933=CARTESIAN_POINT('Origin',(2.0818995585505E-16,3.4,5.7));
#6934=CARTESIAN_POINT('',(0.318956006072958,2.98299632352941,5.7));
#6935=CARTESIAN_POINT('',(0.318956006072958,2.98299632352941,5.7));
#6936=CARTESIAN_POINT('',(-0.318956006072958,2.98299632352941,5.7));
#6937=CARTESIAN_POINT('Origin',(2.0818995585505E-16,3.4,5.7));
#6938=CARTESIAN_POINT('',(-0.318956006072958,2.98299632352941,5.7));
#6939=CARTESIAN_POINT('Origin',(-2.94448637286709,1.7,6.5));
#6940=CARTESIAN_POINT('',(-2.42387259253558,1.76772216571351,6.5));
#6941=CARTESIAN_POINT('',(-2.74282859860853,1.2152741578159,6.5));
#6942=CARTESIAN_POINT('Origin',(0.,0.,6.5));
#6943=CARTESIAN_POINT('Origin',(-2.94448637286709,1.7,6.5));
#6944=CARTESIAN_POINT('Origin',(-2.94448637286709,1.7,5.7));
#6945=CARTESIAN_POINT('',(-2.42387259253558,1.76772216571351,5.7));
#6946=CARTESIAN_POINT('',(-2.42387259253558,1.76772216571351,5.7));
#6947=CARTESIAN_POINT('',(-2.74282859860853,1.2152741578159,5.7));
#6948=CARTESIAN_POINT('Origin',(-2.94448637286709,1.7,5.7));
#6949=CARTESIAN_POINT('',(-2.74282859860853,1.2152741578159,5.7));
#6950=CARTESIAN_POINT('Origin',(-2.94448637286709,-1.7,6.5));
#6951=CARTESIAN_POINT('',(-2.74282859860853,-1.2152741578159,6.5));
#6952=CARTESIAN_POINT('',(-2.42387259253558,-1.76772216571351,6.5));
#6953=CARTESIAN_POINT('Origin',(0.,0.,6.5));
#6954=CARTESIAN_POINT('Origin',(-2.94448637286709,-1.7,6.5));
#6955=CARTESIAN_POINT('Origin',(-2.94448637286709,-1.7,5.7));
#6956=CARTESIAN_POINT('',(-2.74282859860853,-1.2152741578159,5.7));
#6957=CARTESIAN_POINT('',(-2.74282859860853,-1.2152741578159,5.7));
#6958=CARTESIAN_POINT('',(-2.42387259253558,-1.76772216571351,5.7));
#6959=CARTESIAN_POINT('Origin',(-2.94448637286709,-1.7,5.7));
#6960=CARTESIAN_POINT('',(-2.42387259253558,-1.76772216571351,5.7));
#6961=CARTESIAN_POINT('Origin',(2.94448637286709,-1.7,5.7));
#6962=CARTESIAN_POINT('',(2.74282859860853,-1.2152741578159,6.5));
#6963=CARTESIAN_POINT('',(2.74282859860853,-1.2152741578159,5.7));
#6964=CARTESIAN_POINT('',(2.74282859860853,-1.2152741578159,5.7));
#6965=CARTESIAN_POINT('',(2.42387259253558,-1.76772216571351,6.5));
#6966=CARTESIAN_POINT('Origin',(2.94448637286709,-1.7,6.5));
#6967=CARTESIAN_POINT('',(2.42387259253558,-1.76772216571351,5.7));
#6968=CARTESIAN_POINT('',(2.42387259253558,-1.76772216571351,5.7));
#6969=CARTESIAN_POINT('Origin',(2.94448637286709,-1.7,5.7));
#6970=CARTESIAN_POINT('Origin',(2.94448637286709,-1.7,6.5));
#6971=CARTESIAN_POINT('Origin',(0.,0.,6.5));
#6972=CARTESIAN_POINT('Origin',(0.,0.,5.7));
#6973=CARTESIAN_POINT('',(-3.,-3.67394039744206E-16,9.5));
#6974=CARTESIAN_POINT('Origin',(0.,0.,9.5));
#6975=CARTESIAN_POINT('',(-3.,-3.67394039744206E-16,5.7));
#6976=CARTESIAN_POINT('',(-3.,-3.67394039744206E-16,5.7));
#6977=CARTESIAN_POINT('Origin',(0.,0.,5.7));
#6978=CARTESIAN_POINT('Origin',(0.,0.,5.7));
#6979=CARTESIAN_POINT('Origin',(0.,0.,5.7));
#6980=CARTESIAN_POINT('Origin',(0.,0.,5.7));
#6981=CARTESIAN_POINT('Origin',(0.,0.,5.7));
#6982=CARTESIAN_POINT('Origin',(0.,0.,5.7));
#6983=CARTESIAN_POINT('Origin',(0.,0.,5.7));
#6984=CARTESIAN_POINT('Origin',(-6.2456986756515E-16,-3.4,4.9));
#6985=CARTESIAN_POINT('',(-0.275000000000001,-3.4,5.1));
#6986=CARTESIAN_POINT('Origin',(-6.2456986756515E-16,-3.4,5.1));
#6987=CARTESIAN_POINT('',(-0.275000000000001,-3.4,5.7));
#6988=CARTESIAN_POINT('',(-0.275000000000001,-3.4,4.9));
#6989=CARTESIAN_POINT('Origin',(-6.2456986756515E-16,-3.4,5.7));
#6990=CARTESIAN_POINT('Origin',(2.94448637286709,1.7,4.9));
#6991=CARTESIAN_POINT('',(2.66948637286709,1.7,5.1));
#6992=CARTESIAN_POINT('Origin',(2.94448637286709,1.7,5.1));
#6993=CARTESIAN_POINT('',(2.66948637286709,1.7,5.7));
#6994=CARTESIAN_POINT('',(2.66948637286709,1.7,4.9));
#6995=CARTESIAN_POINT('Origin',(2.94448637286709,1.7,5.7));
#6996=CARTESIAN_POINT('Origin',(2.0818995585505E-16,3.4,4.9));
#6997=CARTESIAN_POINT('',(-0.275,3.4,5.1));
#6998=CARTESIAN_POINT('Origin',(2.0818995585505E-16,3.4,5.1));
#6999=CARTESIAN_POINT('',(-0.275,3.4,5.7));
#7000=CARTESIAN_POINT('',(-0.275,3.4,4.9));
#7001=CARTESIAN_POINT('Origin',(2.0818995585505E-16,3.4,5.7));
#7002=CARTESIAN_POINT('Origin',(-2.94448637286709,1.7,4.9));
#7003=CARTESIAN_POINT('',(-3.21948637286709,1.7,5.1));
#7004=CARTESIAN_POINT('Origin',(-2.94448637286709,1.7,5.1));
#7005=CARTESIAN_POINT('',(-3.21948637286709,1.7,5.7));
#7006=CARTESIAN_POINT('',(-3.21948637286709,1.7,4.9));
#7007=CARTESIAN_POINT('Origin',(-2.94448637286709,1.7,5.7));
#7008=CARTESIAN_POINT('Origin',(-2.94448637286709,-1.7,4.9));
#7009=CARTESIAN_POINT('',(-3.21948637286709,-1.7,5.1));
#7010=CARTESIAN_POINT('Origin',(-2.94448637286709,-1.7,5.1));
#7011=CARTESIAN_POINT('',(-3.21948637286709,-1.7,5.7));
#7012=CARTESIAN_POINT('',(-3.21948637286709,-1.7,4.9));
#7013=CARTESIAN_POINT('Origin',(-2.94448637286709,-1.7,5.7));
#7014=CARTESIAN_POINT('Origin',(2.94448637286709,-1.7,4.9));
#7015=CARTESIAN_POINT('',(2.66948637286709,-1.7,5.1));
#7016=CARTESIAN_POINT('Origin',(2.94448637286709,-1.7,5.1));
#7017=CARTESIAN_POINT('',(2.66948637286709,-1.7,5.7));
#7018=CARTESIAN_POINT('',(2.66948637286709,-1.7,4.9));
#7019=CARTESIAN_POINT('Origin',(2.94448637286709,-1.7,5.7));
#7020=CARTESIAN_POINT('Origin',(0.,0.,8.7));
#7021=CARTESIAN_POINT('',(-0.34,-4.163799117101E-17,8.8));
#7022=CARTESIAN_POINT('Origin',(0.,0.,8.8));
#7023=CARTESIAN_POINT('',(-0.34,4.163799117101E-17,9.5));
#7024=CARTESIAN_POINT('',(-0.34,-4.163799117101E-17,8.7));
#7025=CARTESIAN_POINT('Origin',(0.,0.,9.5));
#7026=CARTESIAN_POINT('Origin',(0.,0.,5.));
#7027=CARTESIAN_POINT('',(-2.5,-3.06161699786838E-16,5.1));
#7028=CARTESIAN_POINT('Origin',(0.,0.,5.1));
#7029=CARTESIAN_POINT('',(-2.5,-3.06161699786838E-16,8.8));
#7030=CARTESIAN_POINT('',(-2.5,-3.06161699786838E-16,5.));
#7031=CARTESIAN_POINT('Origin',(0.,0.,8.8));
#7032=CARTESIAN_POINT('Origin',(0.,0.,8.8));
#7033=CARTESIAN_POINT('Origin',(0.,0.,9.5));
#7034=CARTESIAN_POINT('Origin',(0.,0.,5.1));
#7035=CARTESIAN_POINT('',(-4.,-4.89858719658941E-16,5.7));
#7036=CARTESIAN_POINT('Origin',(0.,0.,5.7));
#7037=CARTESIAN_POINT('',(-4.,-4.89858719658941E-16,5.1));
#7038=CARTESIAN_POINT('',(-4.,-4.89858719658941E-16,5.1));
#7039=CARTESIAN_POINT('Origin',(0.,0.,5.1));
#7040=CARTESIAN_POINT('Origin',(0.,0.,5.7));
#7041=CARTESIAN_POINT('Origin',(0.,0.,5.1));
#8389=UNCERTAINTY_MEASURE_WITH_UNIT(LENGTH_MEASURE(0.001),#8429,
'DISTANCE_ACCURACY_VALUE',
'Maximum model space distance between geometric entities at asserted c
onnectivities');
#8402=UNCERTAINTY_MEASURE_WITH_UNIT(LENGTH_MEASURE(0.001),#8429,
'DISTANCE_ACCURACY_VALUE',
'Maximum model space distance between geometric entities at asserted c
onnectivities');
#8415=(
GEOMETRIC_REPRESENTATION_CONTEXT(3)
GLOBAL_UNCERTAINTY_ASSIGNED_CONTEXT((#8389))
GLOBAL_UNIT_ASSIGNED_CONTEXT((#8429,#8431,#8432))
REPRESENTATION_CONTEXT('','3D')
);
#8428=(
GEOMETRIC_REPRESENTATION_CONTEXT(3)
GLOBAL_UNCERTAINTY_ASSIGNED_CONTEXT((#8402))
GLOBAL_UNIT_ASSIGNED_CONTEXT((#8429,#8431,#8432))
REPRESENTATION_CONTEXT('','3D')
);
#8429=(
LENGTH_UNIT()
NAMED_UNIT(*)
SI_UNIT(.CENTI.,.METRE.)
);
#8431=(
NAMED_UNIT(*)
PLANE_ANGLE_UNIT()
SI_UNIT($,.RADIAN.)
);
#8432=(
NAMED_UNIT(*)
SI_UNIT($,.STERADIAN.)
SOLID_ANGLE_UNIT()
);
#8445=SHAPE_DEFINITION_REPRESENTATION(#8470,#8526);
#8470=PRODUCT_DEFINITION_SHAPE('',$,#8552);
#8526=SHAPE_REPRESENTATION('',(#4166),#8415);
#8539=PRODUCT_DEFINITION_CONTEXT('part definition',#8616,'design');
#8552=PRODUCT_DEFINITION('Bonnet','Bonnet',#8577,#8539);
#8577=PRODUCT_DEFINITION_FORMATION('',$,#8630);
#8616=APPLICATION_CONTEXT(
'Core Data for Automotive Mechanical Design Process');
#8617=PRODUCT_CONTEXT('part definition',#8616,'mechanical');
#8630=PRODUCT('Bonnet','Bonnet','Bonnet',(#8617));
#8692=COLOUR_RGB('Sky Blue',0.24,0.69,0.87);
#8693=FILL_AREA_STYLE_COLOUR('',#8692);
#8694=FILL_AREA_STYLE('',(#8693));
#8695=SURFACE_STYLE_FILL_AREA(#8694);
#8696=SURFACE_SIDE_STYLE('',(#8695));
#8697=SURFACE_STYLE_USAGE(.BOTH.,#8696);
#8698=PRESENTATION_STYLE_ASSIGNMENT((#8697));
ENDSEC;
END-ISO-10303-21;
